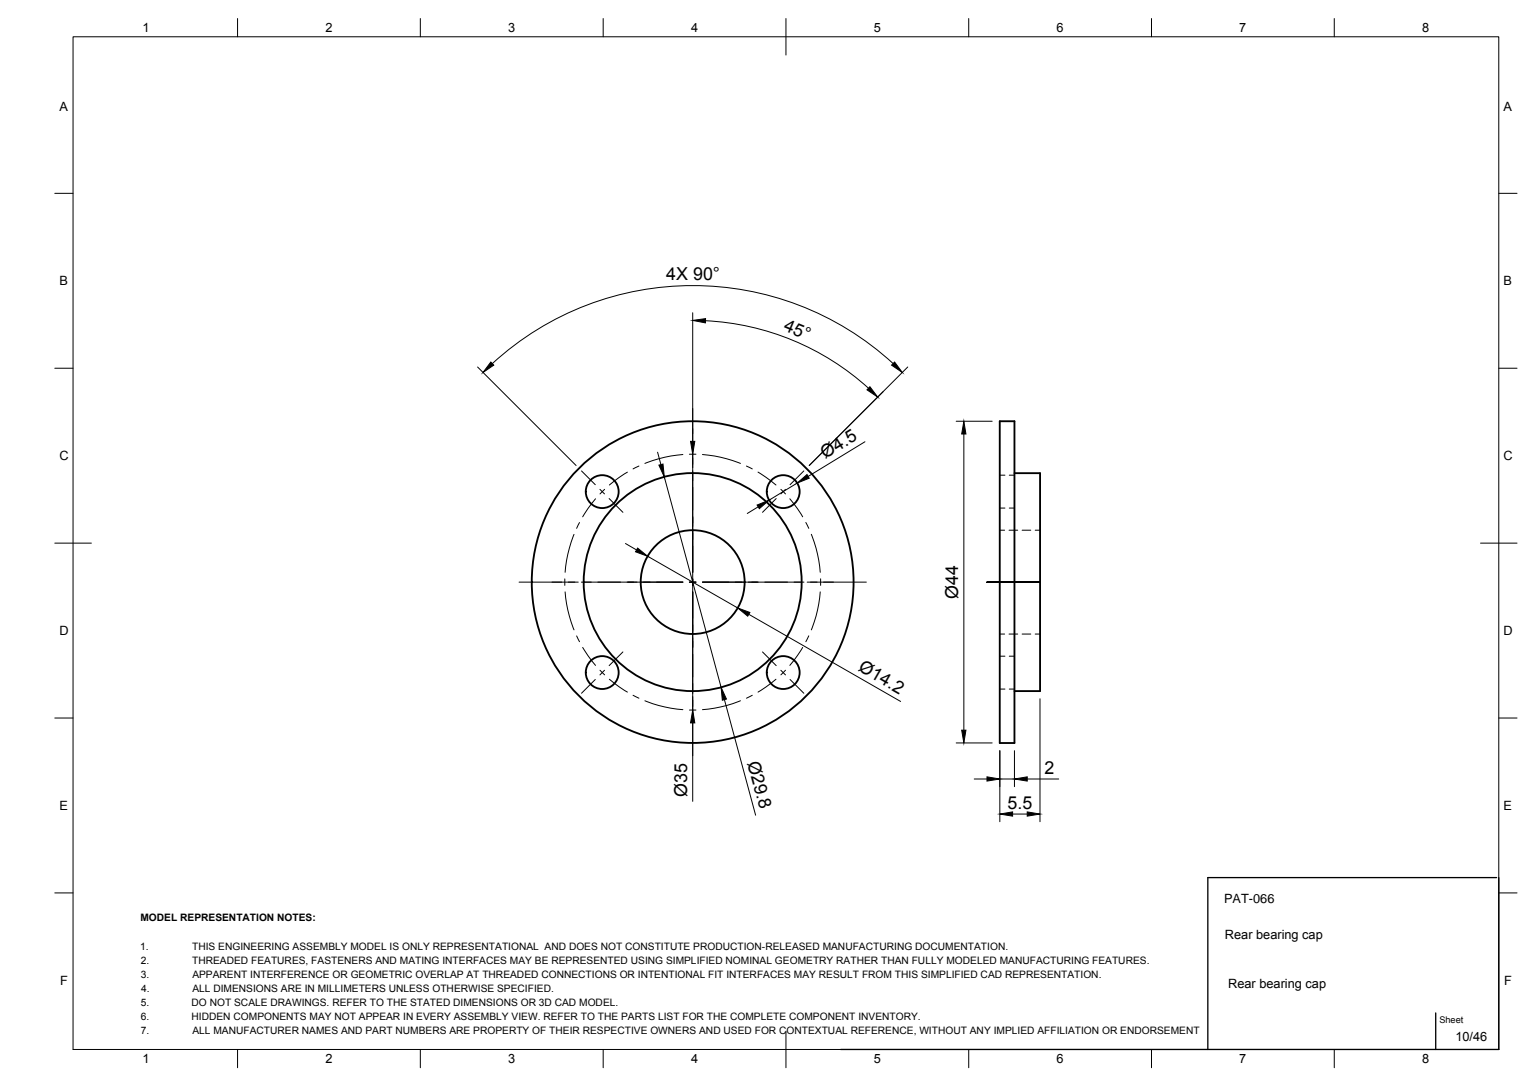
ISO-10303-21;
HEADER;
/* Generated by software containing ST-Developer
 * from STEP Tools, Inc. (www.steptools.com) 
 */

FILE_DESCRIPTION(
/* description */ ('Lever-operated bar clamp (toggle)'),
/* implementation_level */ '2;1');

FILE_NAME(
/* name */ 'Rear bearing cap.step',
/* time_stamp */ '2026-10-28T03:25:02-07:00',
/* author */ (''),
/* organization */ (''),
/* preprocessor_version */ 'ST-DEVELOPER v20.2',
/* originating_system */ 'Autodesk Translation Framework v15.17.0.0',
/* authorisation */ '');

FILE_SCHEMA (('AUTOMOTIVE_DESIGN { 1 0 10303 214 3 1 1 }'));
ENDSEC;

DATA;
#10=MECHANICAL_DESIGN_GEOMETRIC_PRESENTATION_REPRESENTATION('',(#415),#12413);
#339=SHAPE_REPRESENTATION_RELATIONSHIP('SRR','None',#12578,#377);
#377=ADVANCED_BREP_SHAPE_REPRESENTATION('',(#462),#12375);
#415=STYLED_ITEM('',(#12869),#462);
#462=MANIFOLD_SOLID_BREP('Body1',#6574);
#555=FACE_BOUND('',#1429,.T.);
#556=FACE_BOUND('',#1433,.T.);
#557=FACE_BOUND('',#1434,.T.);
#558=FACE_BOUND('',#1435,.T.);
#559=FACE_BOUND('',#1436,.T.);
#560=FACE_BOUND('',#1437,.T.);
#561=FACE_BOUND('',#1439,.T.);
#562=FACE_BOUND('',#1440,.T.);
#563=FACE_BOUND('',#1441,.T.);
#564=FACE_BOUND('',#1442,.T.);
#565=FACE_BOUND('',#1443,.T.);
#692=PLANE('',#7202);
#693=PLANE('',#7209);
#694=PLANE('',#7210);
#962=FACE_OUTER_BOUND('',#1423,.T.);
#963=FACE_OUTER_BOUND('',#1424,.T.);
#964=FACE_OUTER_BOUND('',#1425,.T.);
#965=FACE_OUTER_BOUND('',#1426,.T.);
#966=FACE_OUTER_BOUND('',#1427,.T.);
#967=FACE_OUTER_BOUND('',#1428,.T.);
#968=FACE_OUTER_BOUND('',#1430,.T.);
#969=FACE_OUTER_BOUND('',#1431,.T.);
#970=FACE_OUTER_BOUND('',#1432,.T.);
#971=FACE_OUTER_BOUND('',#1438,.T.);
#1423=EDGE_LOOP('',(#4763,#4764,#4765,#4766));
#1424=EDGE_LOOP('',(#4767,#4768,#4769,#4770));
#1425=EDGE_LOOP('',(#4771,#4772,#4773,#4774));
#1426=EDGE_LOOP('',(#4775,#4776,#4777,#4778));
#1427=EDGE_LOOP('',(#4779,#4780,#4781,#4782));
#1428=EDGE_LOOP('',(#4783));
#1429=EDGE_LOOP('',(#4784));
#1430=EDGE_LOOP('',(#4785,#4786,#4787,#4788));
#1431=EDGE_LOOP('',(#4789,#4790,#4791,#4792));
#1432=EDGE_LOOP('',(#4793));
#1433=EDGE_LOOP('',(#4794));
#1434=EDGE_LOOP('',(#4795));
#1435=EDGE_LOOP('',(#4796));
#1436=EDGE_LOOP('',(#4797));
#1437=EDGE_LOOP('',(#4798));
#1438=EDGE_LOOP('',(#4799));
#1439=EDGE_LOOP('',(#4800));
#1440=EDGE_LOOP('',(#4801));
#1441=EDGE_LOOP('',(#4802));
#1442=EDGE_LOOP('',(#4803));
#1443=EDGE_LOOP('',(#4804));
#1956=LINE('',#10416,#2397);
#1957=LINE('',#10422,#2398);
#1958=LINE('',#10428,#2399);
#1959=LINE('',#10434,#2400);
#1960=LINE('',#10440,#2401);
#1961=LINE('',#10448,#2402);
#1962=LINE('',#10453,#2403);
#2397=VECTOR('',#8299,0.225);
#2398=VECTOR('',#8306,0.225);
#2399=VECTOR('',#8313,0.225);
#2400=VECTOR('',#8320,0.225);
#2401=VECTOR('',#8327,1.49);
#2402=VECTOR('',#8338,0.71);
#2403=VECTOR('',#8343,2.2);
#2799=CIRCLE('',#7188,0.225);
#2800=CIRCLE('',#7189,0.225);
#2801=CIRCLE('',#7191,0.225);
#2802=CIRCLE('',#7192,0.225);
#2803=CIRCLE('',#7194,0.225);
#2804=CIRCLE('',#7195,0.225);
#2805=CIRCLE('',#7197,0.225);
#2806=CIRCLE('',#7198,0.225);
#2807=CIRCLE('',#7200,1.49);
#2808=CIRCLE('',#7201,1.49);
#2809=CIRCLE('',#7203,0.71);
#2810=CIRCLE('',#7205,0.71);
#2811=CIRCLE('',#7207,2.2);
#2812=CIRCLE('',#7208,2.2);
#3188=VERTEX_POINT('',#10413);
#3189=VERTEX_POINT('',#10415);
#3190=VERTEX_POINT('',#10419);
#3191=VERTEX_POINT('',#10421);
#3192=VERTEX_POINT('',#10425);
#3193=VERTEX_POINT('',#10427);
#3194=VERTEX_POINT('',#10431);
#3195=VERTEX_POINT('',#10433);
#3196=VERTEX_POINT('',#10437);
#3197=VERTEX_POINT('',#10439);
#3198=VERTEX_POINT('',#10443);
#3199=VERTEX_POINT('',#10446);
#3200=VERTEX_POINT('',#10450);
#3201=VERTEX_POINT('',#10452);
#3786=EDGE_CURVE('',#3188,#3188,#2799,.T.);
#3787=EDGE_CURVE('',#3188,#3189,#1956,.T.);
#3788=EDGE_CURVE('',#3189,#3189,#2800,.T.);
#3789=EDGE_CURVE('',#3190,#3190,#2801,.T.);
#3790=EDGE_CURVE('',#3190,#3191,#1957,.T.);
#3791=EDGE_CURVE('',#3191,#3191,#2802,.T.);
#3792=EDGE_CURVE('',#3192,#3192,#2803,.T.);
#3793=EDGE_CURVE('',#3192,#3193,#1958,.T.);
#3794=EDGE_CURVE('',#3193,#3193,#2804,.T.);
#3795=EDGE_CURVE('',#3194,#3194,#2805,.T.);
#3796=EDGE_CURVE('',#3194,#3195,#1959,.T.);
#3797=EDGE_CURVE('',#3195,#3195,#2806,.T.);
#3798=EDGE_CURVE('',#3196,#3196,#2807,.T.);
#3799=EDGE_CURVE('',#3196,#3197,#1960,.T.);
#3800=EDGE_CURVE('',#3197,#3197,#2808,.T.);
#3801=EDGE_CURVE('',#3198,#3198,#2809,.T.);
#3802=EDGE_CURVE('',#3199,#3199,#2810,.T.);
#3803=EDGE_CURVE('',#3199,#3198,#1961,.T.);
#3804=EDGE_CURVE('',#3200,#3200,#2811,.T.);
#3805=EDGE_CURVE('',#3200,#3201,#1962,.T.);
#3806=EDGE_CURVE('',#3201,#3201,#2812,.T.);
#4763=ORIENTED_EDGE('',*,*,#3786,.F.);
#4764=ORIENTED_EDGE('',*,*,#3787,.T.);
#4765=ORIENTED_EDGE('',*,*,#3788,.F.);
#4766=ORIENTED_EDGE('',*,*,#3787,.F.);
#4767=ORIENTED_EDGE('',*,*,#3789,.F.);
#4768=ORIENTED_EDGE('',*,*,#3790,.T.);
#4769=ORIENTED_EDGE('',*,*,#3791,.F.);
#4770=ORIENTED_EDGE('',*,*,#3790,.F.);
#4771=ORIENTED_EDGE('',*,*,#3792,.F.);
#4772=ORIENTED_EDGE('',*,*,#3793,.T.);
#4773=ORIENTED_EDGE('',*,*,#3794,.F.);
#4774=ORIENTED_EDGE('',*,*,#3793,.F.);
#4775=ORIENTED_EDGE('',*,*,#3795,.F.);
#4776=ORIENTED_EDGE('',*,*,#3796,.T.);
#4777=ORIENTED_EDGE('',*,*,#3797,.F.);
#4778=ORIENTED_EDGE('',*,*,#3796,.F.);
#4779=ORIENTED_EDGE('',*,*,#3798,.F.);
#4780=ORIENTED_EDGE('',*,*,#3799,.T.);
#4781=ORIENTED_EDGE('',*,*,#3800,.T.);
#4782=ORIENTED_EDGE('',*,*,#3799,.F.);
#4783=ORIENTED_EDGE('',*,*,#3800,.F.);
#4784=ORIENTED_EDGE('',*,*,#3801,.F.);
#4785=ORIENTED_EDGE('',*,*,#3802,.F.);
#4786=ORIENTED_EDGE('',*,*,#3803,.T.);
#4787=ORIENTED_EDGE('',*,*,#3801,.T.);
#4788=ORIENTED_EDGE('',*,*,#3803,.F.);
#4789=ORIENTED_EDGE('',*,*,#3804,.F.);
#4790=ORIENTED_EDGE('',*,*,#3805,.T.);
#4791=ORIENTED_EDGE('',*,*,#3806,.T.);
#4792=ORIENTED_EDGE('',*,*,#3805,.F.);
#4793=ORIENTED_EDGE('',*,*,#3804,.T.);
#4794=ORIENTED_EDGE('',*,*,#3802,.T.);
#4795=ORIENTED_EDGE('',*,*,#3797,.T.);
#4796=ORIENTED_EDGE('',*,*,#3794,.T.);
#4797=ORIENTED_EDGE('',*,*,#3791,.T.);
#4798=ORIENTED_EDGE('',*,*,#3788,.T.);
#4799=ORIENTED_EDGE('',*,*,#3806,.F.);
#4800=ORIENTED_EDGE('',*,*,#3798,.T.);
#4801=ORIENTED_EDGE('',*,*,#3795,.T.);
#4802=ORIENTED_EDGE('',*,*,#3792,.T.);
#4803=ORIENTED_EDGE('',*,*,#3789,.T.);
#4804=ORIENTED_EDGE('',*,*,#3786,.T.);
#6066=CYLINDRICAL_SURFACE('',#7187,0.225);
#6067=CYLINDRICAL_SURFACE('',#7190,0.225);
#6068=CYLINDRICAL_SURFACE('',#7193,0.225);
#6069=CYLINDRICAL_SURFACE('',#7196,0.225);
#6070=CYLINDRICAL_SURFACE('',#7199,1.49);
#6071=CYLINDRICAL_SURFACE('',#7204,0.71);
#6072=CYLINDRICAL_SURFACE('',#7206,2.2);
#6237=ADVANCED_FACE('',(#962),#6066,.F.);
#6238=ADVANCED_FACE('',(#963),#6067,.F.);
#6239=ADVANCED_FACE('',(#964),#6068,.F.);
#6240=ADVANCED_FACE('',(#965),#6069,.F.);
#6241=ADVANCED_FACE('',(#966),#6070,.T.);
#6242=ADVANCED_FACE('',(#967,#555),#692,.F.);
#6243=ADVANCED_FACE('',(#968),#6071,.F.);
#6244=ADVANCED_FACE('',(#969),#6072,.T.);
#6245=ADVANCED_FACE('',(#970,#556,#557,#558,#559,#560),#693,.T.);
#6246=ADVANCED_FACE('',(#971,#561,#562,#563,#564,#565),#694,.F.);
#6574=CLOSED_SHELL('',(#6237,#6238,#6239,#6240,#6241,#6242,#6243,#6244,
#6245,#6246));
#7186=AXIS2_PLACEMENT_3D('',#10411,#8293,#8294);
#7187=AXIS2_PLACEMENT_3D('',#10412,#8295,#8296);
#7188=AXIS2_PLACEMENT_3D('',#10414,#8297,#8298);
#7189=AXIS2_PLACEMENT_3D('',#10417,#8300,#8301);
#7190=AXIS2_PLACEMENT_3D('',#10418,#8302,#8303);
#7191=AXIS2_PLACEMENT_3D('',#10420,#8304,#8305);
#7192=AXIS2_PLACEMENT_3D('',#10423,#8307,#8308);
#7193=AXIS2_PLACEMENT_3D('',#10424,#8309,#8310);
#7194=AXIS2_PLACEMENT_3D('',#10426,#8311,#8312);
#7195=AXIS2_PLACEMENT_3D('',#10429,#8314,#8315);
#7196=AXIS2_PLACEMENT_3D('',#10430,#8316,#8317);
#7197=AXIS2_PLACEMENT_3D('',#10432,#8318,#8319);
#7198=AXIS2_PLACEMENT_3D('',#10435,#8321,#8322);
#7199=AXIS2_PLACEMENT_3D('',#10436,#8323,#8324);
#7200=AXIS2_PLACEMENT_3D('',#10438,#8325,#8326);
#7201=AXIS2_PLACEMENT_3D('',#10441,#8328,#8329);
#7202=AXIS2_PLACEMENT_3D('',#10442,#8330,#8331);
#7203=AXIS2_PLACEMENT_3D('',#10444,#8332,#8333);
#7204=AXIS2_PLACEMENT_3D('',#10445,#8334,#8335);
#7205=AXIS2_PLACEMENT_3D('',#10447,#8336,#8337);
#7206=AXIS2_PLACEMENT_3D('',#10449,#8339,#8340);
#7207=AXIS2_PLACEMENT_3D('',#10451,#8341,#8342);
#7208=AXIS2_PLACEMENT_3D('',#10454,#8344,#8345);
#7209=AXIS2_PLACEMENT_3D('',#10455,#8346,#8347);
#7210=AXIS2_PLACEMENT_3D('',#10456,#8348,#8349);
#8293=DIRECTION('axis',(0.,0.,1.));
#8294=DIRECTION('refdir',(1.,0.,0.));
#8295=DIRECTION('center_axis',(0.,1.,0.));
#8296=DIRECTION('ref_axis',(1.,0.,0.));
#8297=DIRECTION('center_axis',(0.,1.,0.));
#8298=DIRECTION('ref_axis',(1.,0.,0.));
#8299=DIRECTION('',(0.,1.,0.));
#8300=DIRECTION('center_axis',(0.,-1.,0.));
#8301=DIRECTION('ref_axis',(1.,0.,0.));
#8302=DIRECTION('center_axis',(0.,1.,0.));
#8303=DIRECTION('ref_axis',(1.,0.,0.));
#8304=DIRECTION('center_axis',(0.,1.,0.));
#8305=DIRECTION('ref_axis',(1.,0.,0.));
#8306=DIRECTION('',(0.,1.,0.));
#8307=DIRECTION('center_axis',(0.,-1.,0.));
#8308=DIRECTION('ref_axis',(1.,0.,0.));
#8309=DIRECTION('center_axis',(0.,1.,0.));
#8310=DIRECTION('ref_axis',(1.,0.,0.));
#8311=DIRECTION('center_axis',(0.,1.,0.));
#8312=DIRECTION('ref_axis',(1.,0.,0.));
#8313=DIRECTION('',(0.,1.,0.));
#8314=DIRECTION('center_axis',(0.,-1.,0.));
#8315=DIRECTION('ref_axis',(1.,0.,0.));
#8316=DIRECTION('center_axis',(0.,1.,0.));
#8317=DIRECTION('ref_axis',(1.,0.,0.));
#8318=DIRECTION('center_axis',(0.,1.,0.));
#8319=DIRECTION('ref_axis',(1.,0.,0.));
#8320=DIRECTION('',(0.,1.,0.));
#8321=DIRECTION('center_axis',(0.,-1.,0.));
#8322=DIRECTION('ref_axis',(1.,0.,0.));
#8323=DIRECTION('center_axis',(0.,1.,0.));
#8324=DIRECTION('ref_axis',(1.,0.,0.));
#8325=DIRECTION('center_axis',(0.,1.,0.));
#8326=DIRECTION('ref_axis',(1.,0.,0.));
#8327=DIRECTION('',(0.,-1.,0.));
#8328=DIRECTION('center_axis',(0.,1.,0.));
#8329=DIRECTION('ref_axis',(1.,0.,0.));
#8330=DIRECTION('center_axis',(0.,1.,0.));
#8331=DIRECTION('ref_axis',(1.,0.,0.));
#8332=DIRECTION('center_axis',(0.,-1.,0.));
#8333=DIRECTION('ref_axis',(1.,0.,0.));
#8334=DIRECTION('center_axis',(0.,1.,0.));
#8335=DIRECTION('ref_axis',(1.,0.,0.));
#8336=DIRECTION('center_axis',(0.,-1.,0.));
#8337=DIRECTION('ref_axis',(1.,0.,0.));
#8338=DIRECTION('',(0.,-1.,0.));
#8339=DIRECTION('center_axis',(0.,1.,0.));
#8340=DIRECTION('ref_axis',(1.,0.,0.));
#8341=DIRECTION('center_axis',(0.,1.,0.));
#8342=DIRECTION('ref_axis',(1.,0.,0.));
#8343=DIRECTION('',(0.,-1.,0.));
#8344=DIRECTION('center_axis',(0.,1.,0.));
#8345=DIRECTION('ref_axis',(1.,0.,0.));
#8346=DIRECTION('center_axis',(0.,1.,0.));
#8347=DIRECTION('ref_axis',(1.,0.,0.));
#8348=DIRECTION('center_axis',(0.,1.,0.));
#8349=DIRECTION('ref_axis',(1.,0.,0.));
#10411=CARTESIAN_POINT('',(0.,0.,0.));
#10412=CARTESIAN_POINT('Origin',(-5.23743686707646,0.7,9.76256313292354));
#10413=CARTESIAN_POINT('',(-5.46243686707646,0.8,9.76256313292354));
#10414=CARTESIAN_POINT('Origin',(-5.23743686707646,0.8,9.76256313292354));
#10415=CARTESIAN_POINT('',(-5.46243686707646,1.,9.76256313292354));
#10416=CARTESIAN_POINT('',(-5.46243686707646,0.7,9.76256313292354));
#10417=CARTESIAN_POINT('Origin',(-5.23743686707646,1.,9.76256313292354));
#10418=CARTESIAN_POINT('Origin',(-5.23743686707646,0.7,12.2374368670765));
#10419=CARTESIAN_POINT('',(-5.46243686707646,0.8,12.2374368670765));
#10420=CARTESIAN_POINT('Origin',(-5.23743686707646,0.8,12.2374368670765));
#10421=CARTESIAN_POINT('',(-5.46243686707646,1.,12.2374368670765));
#10422=CARTESIAN_POINT('',(-5.46243686707646,0.7,12.2374368670765));
#10423=CARTESIAN_POINT('Origin',(-5.23743686707646,1.,12.2374368670765));
#10424=CARTESIAN_POINT('Origin',(-2.76256313292354,0.7,12.2374368670765));
#10425=CARTESIAN_POINT('',(-2.98756313292354,0.8,12.2374368670765));
#10426=CARTESIAN_POINT('Origin',(-2.76256313292354,0.8,12.2374368670765));
#10427=CARTESIAN_POINT('',(-2.98756313292354,1.,12.2374368670765));
#10428=CARTESIAN_POINT('',(-2.98756313292354,0.7,12.2374368670765));
#10429=CARTESIAN_POINT('Origin',(-2.76256313292354,1.,12.2374368670765));
#10430=CARTESIAN_POINT('Origin',(-2.76256313292354,0.7,9.76256313292354));
#10431=CARTESIAN_POINT('',(-2.98756313292354,0.8,9.76256313292354));
#10432=CARTESIAN_POINT('Origin',(-2.76256313292354,0.8,9.76256313292354));
#10433=CARTESIAN_POINT('',(-2.98756313292354,1.,9.76256313292354));
#10434=CARTESIAN_POINT('',(-2.98756313292354,0.7,9.76256313292354));
#10435=CARTESIAN_POINT('Origin',(-2.76256313292354,1.,9.76256313292354));
#10436=CARTESIAN_POINT('Origin',(-4.,0.45,11.));
#10437=CARTESIAN_POINT('',(-5.49,0.8,11.));
#10438=CARTESIAN_POINT('Origin',(-4.,0.8,11.));
#10439=CARTESIAN_POINT('',(-5.49,0.45,11.));
#10440=CARTESIAN_POINT('',(-5.49,0.45,11.));
#10441=CARTESIAN_POINT('Origin',(-4.,0.45,11.));
#10442=CARTESIAN_POINT('Origin',(-4.,0.45,11.));
#10443=CARTESIAN_POINT('',(-4.71,0.45,11.));
#10444=CARTESIAN_POINT('Origin',(-4.,0.45,11.));
#10445=CARTESIAN_POINT('Origin',(-4.,0.8,11.));
#10446=CARTESIAN_POINT('',(-4.71,1.,11.));
#10447=CARTESIAN_POINT('Origin',(-4.,1.,11.));
#10448=CARTESIAN_POINT('',(-4.71,0.8,11.));
#10449=CARTESIAN_POINT('Origin',(-4.,0.8,11.));
#10450=CARTESIAN_POINT('',(-6.2,1.,11.));
#10451=CARTESIAN_POINT('Origin',(-4.,1.,11.));
#10452=CARTESIAN_POINT('',(-6.2,0.8,11.));
#10453=CARTESIAN_POINT('',(-6.2,0.8,11.));
#10454=CARTESIAN_POINT('Origin',(-4.,0.8,11.));
#10455=CARTESIAN_POINT('Origin',(-4.,1.,11.));
#10456=CARTESIAN_POINT('Origin',(-4.,0.8,11.));
#12329=UNCERTAINTY_MEASURE_WITH_UNIT(LENGTH_MEASURE(0.001),#12414,
'DISTANCE_ACCURACY_VALUE',
'Maximum model space distance between geometric entities at asserted c
onnectivities');
#12367=UNCERTAINTY_MEASURE_WITH_UNIT(LENGTH_MEASURE(0.001),#12414,
'DISTANCE_ACCURACY_VALUE',
'Maximum model space distance between geometric entities at asserted c
onnectivities');
#12375=(
GEOMETRIC_REPRESENTATION_CONTEXT(3)
GLOBAL_UNCERTAINTY_ASSIGNED_CONTEXT((#12329))
GLOBAL_UNIT_ASSIGNED_CONTEXT((#12414,#12416,#12417))
REPRESENTATION_CONTEXT('','3D')
);
#12413=(
GEOMETRIC_REPRESENTATION_CONTEXT(3)
GLOBAL_UNCERTAINTY_ASSIGNED_CONTEXT((#12367))
GLOBAL_UNIT_ASSIGNED_CONTEXT((#12414,#12416,#12417))
REPRESENTATION_CONTEXT('','3D')
);
#12414=(
LENGTH_UNIT()
NAMED_UNIT(*)
SI_UNIT(.CENTI.,.METRE.)
);
#12416=(
NAMED_UNIT(*)
PLANE_ANGLE_UNIT()
SI_UNIT($,.RADIAN.)
);
#12417=(
NAMED_UNIT(*)
SI_UNIT($,.STERADIAN.)
SOLID_ANGLE_UNIT()
);
#12425=SHAPE_DEFINITION_REPRESENTATION(#12470,#12578);
#12470=PRODUCT_DEFINITION_SHAPE('',$,#12624);
#12578=SHAPE_REPRESENTATION('',(#7186),#12375);
#12616=PRODUCT_DEFINITION_CONTEXT('part definition',#12753,'design');
#12624=PRODUCT_DEFINITION('Rear bearing cap','Rear bearing cap',#12669,
#12616);
#12669=PRODUCT_DEFINITION_FORMATION('',$,#12762);
#12753=APPLICATION_CONTEXT(
'Core Data for Automotive Mechanical Design Process');
#12754=PRODUCT_CONTEXT('part definition',#12753,'mechanical');
#12762=PRODUCT('Rear bearing cap','Rear bearing cap','Rear bearing cap',
(#12754));
#12863=COLOUR_RGB('Grey',0.48,0.52,0.57);
#12864=FILL_AREA_STYLE_COLOUR('',#12863);
#12865=FILL_AREA_STYLE('',(#12864));
#12866=SURFACE_STYLE_FILL_AREA(#12865);
#12867=SURFACE_SIDE_STYLE('',(#12866));
#12868=SURFACE_STYLE_USAGE(.BOTH.,#12867);
#12869=PRESENTATION_STYLE_ASSIGNMENT((#12868));
ENDSEC;
END-ISO-10303-21;
